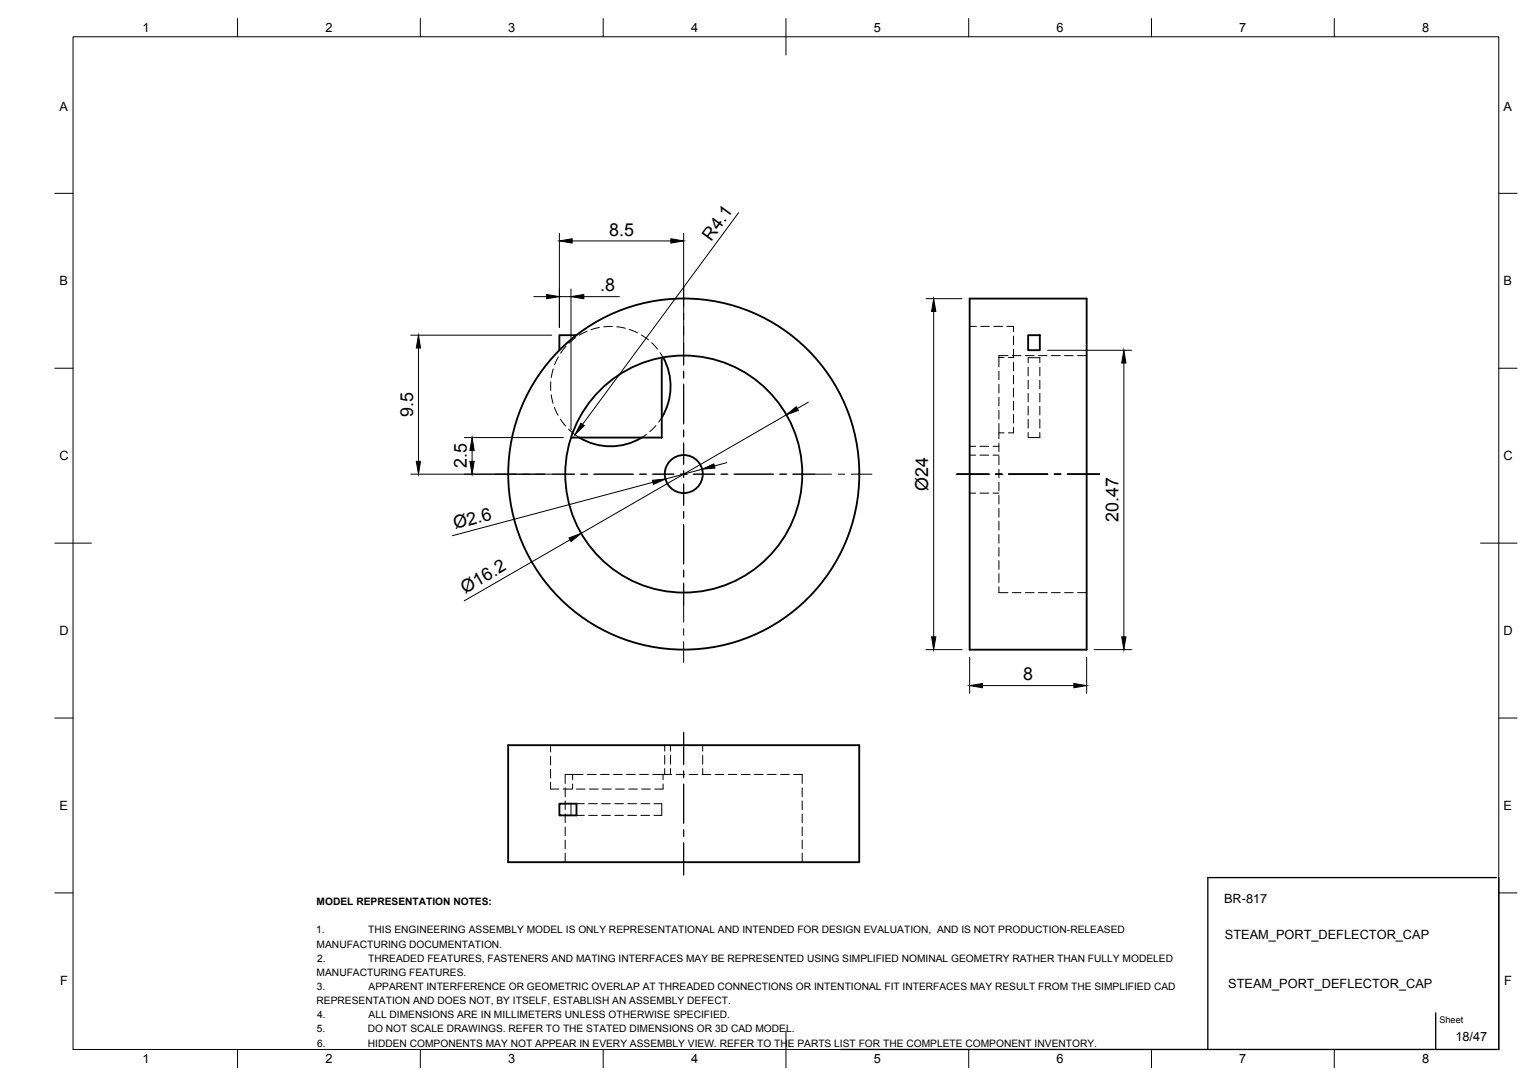
ISO-10303-21;
HEADER;
FILE_DESCRIPTION((''),'2;1');
FILE_NAME('STEAM_PORT_DEFLECTOR_CAP.step','2026-10-01T22:07:29-07:00',(''),(''),'','','');
FILE_SCHEMA (('AUTOMOTIVE_DESIGN { 1 0 10303 214 3 1 1 }'));
ENDSEC;
DATA;
#10=MECHANICAL_DESIGN_GEOMETRIC_PRESENTATION_REPRESENTATION('',(#552),#15484);
#482=SHAPE_REPRESENTATION_RELATIONSHIP('SRR','None',#15631,#517) ;
#517=ADVANCED_BREP_SHAPE_REPRESENTATION('',(#594),#15455) ;
#552=STYLED_ITEM('',(#15836),#594) ;
#594=MANIFOLD_SOLID_BREP('STEAM_PORT_DEFLECTOR_CAP',#8261) ;
#663=CYLINDRICAL_SURFACE('',#8912,0.13) ;
#664=CYLINDRICAL_SURFACE('',#8918,0.41) ;
#665=CYLINDRICAL_SURFACE('',#8922,0.81) ;
#666=CYLINDRICAL_SURFACE('',#8929,1.2) ;
#853=FACE_BOUND('',#2043,.T.) ;
#854=FACE_BOUND('',#2045,.T.) ;
#855=FACE_BOUND('',#2047,.T.) ;
#856=FACE_BOUND('',#2048,.T.) ;
#857=FACE_BOUND('',#2050,.T.) ;
#858=FACE_BOUND('',#2052,.T.) ;
#960=CIRCLE('',#8902,1.2) ;
#961=CIRCLE('',#8905,1.2) ;
#962=CIRCLE('',#8907,0.81) ;
#963=CIRCLE('',#8909,0.81) ;
#964=CIRCLE('',#8913,0.13) ;
#965=CIRCLE('',#8914,0.13) ;
#966=CIRCLE('',#8916,0.81) ;
#967=CIRCLE('',#8917,0.41) ;
#968=CIRCLE('',#8919,0.41) ;
#969=CIRCLE('',#8920,0.41) ;
#970=CIRCLE('',#8921,0.41) ;
#971=CIRCLE('',#8923,0.81) ;
#972=CIRCLE('',#8924,0.81) ;
#973=CIRCLE('',#8925,0.81) ;
#974=CIRCLE('',#8928,1.2) ;
#975=CIRCLE('',#8930,1.2) ;
#1488=FACE_OUTER_BOUND('',#2031,.T.) ;
#1489=FACE_OUTER_BOUND('',#2032,.T.) ;
#1490=FACE_OUTER_BOUND('',#2033,.T.) ;
#1491=FACE_OUTER_BOUND('',#2034,.T.) ;
#1492=FACE_OUTER_BOUND('',#2035,.T.) ;
#1493=FACE_OUTER_BOUND('',#2036,.T.) ;
#1494=FACE_OUTER_BOUND('',#2037,.T.) ;
#1495=FACE_OUTER_BOUND('',#2038,.T.) ;
#1496=FACE_OUTER_BOUND('',#2039,.T.) ;
#1497=FACE_OUTER_BOUND('',#2040,.T.) ;
#1498=FACE_OUTER_BOUND('',#2041,.T.) ;
#1499=FACE_OUTER_BOUND('',#2042,.T.) ;
#1500=FACE_OUTER_BOUND('',#2044,.T.) ;
#1501=FACE_OUTER_BOUND('',#2046,.T.) ;
#1502=FACE_OUTER_BOUND('',#2049,.T.) ;
#1503=FACE_OUTER_BOUND('',#2051,.T.) ;
#2031=EDGE_LOOP('',(#5779,#5780,#5781,#5782)) ;
#2032=EDGE_LOOP('',(#5783,#5784,#5785)) ;
#2033=EDGE_LOOP('',(#5786,#5787,#5788,#5789)) ;
#2034=EDGE_LOOP('',(#5790,#5791,#5792)) ;
#2035=EDGE_LOOP('',(#5793,#5794,#5795)) ;
#2036=EDGE_LOOP('',(#5796,#5797,#5798)) ;
#2037=EDGE_LOOP('',(#5799,#5800,#5801,#5802)) ;
#2038=EDGE_LOOP('',(#5803,#5804,#5805,#5806)) ;
#2039=EDGE_LOOP('',(#5807,#5808,#5809,#5810)) ;
#2040=EDGE_LOOP('',(#5811,#5812)) ;
#2041=EDGE_LOOP('',(#5813,#5814,#5815,#5816,#5817,#5818,#5819,#5820)) ;
#2042=EDGE_LOOP('',(#5821,#5822,#5823,#5824,#5825,#5826,#5827,#5828)) ;
#2043=EDGE_LOOP('',(#5829,#5830,#5831,#5832)) ;
#2044=EDGE_LOOP('',(#5833,#5834,#5835,#5836)) ;
#2045=EDGE_LOOP('',(#5837)) ;
#2046=EDGE_LOOP('',(#5838)) ;
#2047=EDGE_LOOP('',(#5839)) ;
#2048=EDGE_LOOP('',(#5840)) ;
#2049=EDGE_LOOP('',(#5841,#5842,#5843,#5844)) ;
#2050=EDGE_LOOP('',(#5845,#5846,#5847,#5848)) ;
#2051=EDGE_LOOP('',(#5849)) ;
#2052=EDGE_LOOP('',(#5850)) ;
#2618=LINE('',#13453,#3092) ;
#2619=LINE('',#13455,#3093) ;
#2620=LINE('',#13457,#3094) ;
#2621=LINE('',#13458,#3095) ;
#2622=LINE('',#13464,#3096) ;
#2623=LINE('',#13465,#3097) ;
#2624=LINE('',#13468,#3098) ;
#2625=LINE('',#13470,#3099) ;
#2626=LINE('',#13471,#3100) ;
#2627=LINE('',#13475,#3101) ;
#2628=LINE('',#13479,#3102) ;
#2629=LINE('',#13483,#3103) ;
#2630=LINE('',#13485,#3104) ;
#2631=LINE('',#13487,#3105) ;
#2632=LINE('',#13492,#3106) ;
#2633=LINE('',#13501,#3107) ;
#2634=LINE('',#13505,#3108) ;
#2635=LINE('',#13509,#3109) ;
#2636=LINE('',#13514,#3110) ;
#2637=LINE('',#13523,#3111) ;
#3092=VECTOR('',#10541,1.) ;
#3093=VECTOR('',#10542,1.) ;
#3094=VECTOR('',#10543,1.) ;
#3095=VECTOR('',#10544,1.) ;
#3096=VECTOR('',#10549,1.) ;
#3097=VECTOR('',#10550,1.) ;
#3098=VECTOR('',#10553,1.) ;
#3099=VECTOR('',#10554,1.) ;
#3100=VECTOR('',#10555,1.) ;
#3101=VECTOR('',#10560,1.) ;
#3102=VECTOR('',#10565,1.) ;
#3103=VECTOR('',#10570,1.) ;
#3104=VECTOR('',#10573,1.) ;
#3105=VECTOR('',#10576,1.) ;
#3106=VECTOR('',#10581,0.13) ;
#3107=VECTOR('',#10592,1.) ;
#3108=VECTOR('',#10595,0.41) ;
#3109=VECTOR('',#10600,1.) ;
#3110=VECTOR('',#10605,0.81) ;
#3111=VECTOR('',#10618,1.2) ;
#3557=VERTEX_POINT('',#13451) ;
#3558=VERTEX_POINT('',#13452) ;
#3559=VERTEX_POINT('',#13454) ;
#3560=VERTEX_POINT('',#13456) ;
#3561=VERTEX_POINT('',#13460) ;
#3562=VERTEX_POINT('',#13461) ;
#3563=VERTEX_POINT('',#13463) ;
#3564=VERTEX_POINT('',#13467) ;
#3565=VERTEX_POINT('',#13469) ;
#3566=VERTEX_POINT('',#13473) ;
#3567=VERTEX_POINT('',#13477) ;
#3568=VERTEX_POINT('',#13481) ;
#3569=VERTEX_POINT('',#13489) ;
#3570=VERTEX_POINT('',#13491) ;
#3571=VERTEX_POINT('',#13495) ;
#3572=VERTEX_POINT('',#13496) ;
#3573=VERTEX_POINT('',#13500) ;
#3574=VERTEX_POINT('',#13502) ;
#3575=VERTEX_POINT('',#13504) ;
#3576=VERTEX_POINT('',#13507) ;
#3577=VERTEX_POINT('',#13511) ;
#3578=VERTEX_POINT('',#13513) ;
#3579=VERTEX_POINT('',#13519) ;
#3580=VERTEX_POINT('',#13522) ;
#4394=EDGE_CURVE('',#3557,#3558,#2618,.T.) ;
#4395=EDGE_CURVE('',#3559,#3557,#2619,.T.) ;
#4396=EDGE_CURVE('',#3560,#3559,#2620,.T.) ;
#4397=EDGE_CURVE('',#3558,#3560,#2621,.T.) ;
#4398=EDGE_CURVE('',#3561,#3562,#960,.T.) ;
#4399=EDGE_CURVE('',#3561,#3563,#2622,.T.) ;
#4400=EDGE_CURVE('',#3563,#3562,#2623,.T.) ;
#4401=EDGE_CURVE('',#3564,#3561,#2624,.T.) ;
#4402=EDGE_CURVE('',#3565,#3564,#2625,.T.) ;
#4403=EDGE_CURVE('',#3563,#3565,#2626,.T.) ;
#4404=EDGE_CURVE('',#3566,#3564,#961,.T.) ;
#4405=EDGE_CURVE('',#3566,#3565,#2627,.T.) ;
#4406=EDGE_CURVE('',#3567,#3557,#962,.T.) ;
#4407=EDGE_CURVE('',#3567,#3559,#2628,.T.) ;
#4408=EDGE_CURVE('',#3558,#3568,#963,.T.) ;
#4409=EDGE_CURVE('',#3560,#3568,#2629,.T.) ;
#4410=EDGE_CURVE('',#3568,#3567,#2630,.T.) ;
#4411=EDGE_CURVE('',#3562,#3566,#2631,.T.) ;
#4412=EDGE_CURVE('',#3569,#3569,#964,.T.) ;
#4413=EDGE_CURVE('',#3569,#3570,#2632,.T.) ;
#4414=EDGE_CURVE('',#3570,#3570,#965,.T.) ;
#4415=EDGE_CURVE('',#3571,#3572,#966,.T.) ;
#4416=EDGE_CURVE('',#3572,#3571,#967,.T.) ;
#4417=EDGE_CURVE('',#3573,#3571,#2633,.T.) ;
#4418=EDGE_CURVE('',#3574,#3573,#968,.T.) ;
#4419=EDGE_CURVE('',#3574,#3575,#2634,.T.) ;
#4420=EDGE_CURVE('',#3575,#3575,#969,.T.) ;
#4421=EDGE_CURVE('',#3576,#3574,#970,.T.) ;
#4422=EDGE_CURVE('',#3572,#3576,#2635,.T.) ;
#4423=EDGE_CURVE('',#3577,#3577,#971,.T.) ;
#4424=EDGE_CURVE('',#3577,#3578,#2636,.T.) ;
#4425=EDGE_CURVE('',#3573,#3578,#972,.T.) ;
#4426=EDGE_CURVE('',#3578,#3576,#973,.T.) ;
#4427=EDGE_CURVE('',#3579,#3579,#974,.T.) ;
#4428=EDGE_CURVE('',#3579,#3580,#2637,.T.) ;
#4429=EDGE_CURVE('',#3580,#3580,#975,.T.) ;
#5779=ORIENTED_EDGE('',*,*,#4394,.F.) ;
#5780=ORIENTED_EDGE('',*,*,#4395,.F.) ;
#5781=ORIENTED_EDGE('',*,*,#4396,.F.) ;
#5782=ORIENTED_EDGE('',*,*,#4397,.F.) ;
#5783=ORIENTED_EDGE('',*,*,#4398,.F.) ;
#5784=ORIENTED_EDGE('',*,*,#4399,.T.) ;
#5785=ORIENTED_EDGE('',*,*,#4400,.T.) ;
#5786=ORIENTED_EDGE('',*,*,#4401,.F.) ;
#5787=ORIENTED_EDGE('',*,*,#4402,.F.) ;
#5788=ORIENTED_EDGE('',*,*,#4403,.F.) ;
#5789=ORIENTED_EDGE('',*,*,#4399,.F.) ;
#5790=ORIENTED_EDGE('',*,*,#4404,.F.) ;
#5791=ORIENTED_EDGE('',*,*,#4405,.T.) ;
#5792=ORIENTED_EDGE('',*,*,#4402,.T.) ;
#5793=ORIENTED_EDGE('',*,*,#4406,.F.) ;
#5794=ORIENTED_EDGE('',*,*,#4407,.T.) ;
#5795=ORIENTED_EDGE('',*,*,#4395,.T.) ;
#5796=ORIENTED_EDGE('',*,*,#4408,.F.) ;
#5797=ORIENTED_EDGE('',*,*,#4397,.T.) ;
#5798=ORIENTED_EDGE('',*,*,#4409,.T.) ;
#5799=ORIENTED_EDGE('',*,*,#4410,.F.) ;
#5800=ORIENTED_EDGE('',*,*,#4409,.F.) ;
#5801=ORIENTED_EDGE('',*,*,#4396,.T.) ;
#5802=ORIENTED_EDGE('',*,*,#4407,.F.) ;
#5803=ORIENTED_EDGE('',*,*,#4411,.F.) ;
#5804=ORIENTED_EDGE('',*,*,#4400,.F.) ;
#5805=ORIENTED_EDGE('',*,*,#4403,.T.) ;
#5806=ORIENTED_EDGE('',*,*,#4405,.F.) ;
#5807=ORIENTED_EDGE('',*,*,#4412,.F.) ;
#5808=ORIENTED_EDGE('',*,*,#4413,.T.) ;
#5809=ORIENTED_EDGE('',*,*,#4414,.F.) ;
#5810=ORIENTED_EDGE('',*,*,#4413,.F.) ;
#5811=ORIENTED_EDGE('',*,*,#4415,.F.) ;
#5812=ORIENTED_EDGE('',*,*,#4416,.F.) ;
#5813=ORIENTED_EDGE('',*,*,#4417,.F.) ;
#5814=ORIENTED_EDGE('',*,*,#4418,.F.) ;
#5815=ORIENTED_EDGE('',*,*,#4419,.T.) ;
#5816=ORIENTED_EDGE('',*,*,#4420,.F.) ;
#5817=ORIENTED_EDGE('',*,*,#4419,.F.) ;
#5818=ORIENTED_EDGE('',*,*,#4421,.F.) ;
#5819=ORIENTED_EDGE('',*,*,#4422,.F.) ;
#5820=ORIENTED_EDGE('',*,*,#4416,.T.) ;
#5821=ORIENTED_EDGE('',*,*,#4423,.F.) ;
#5822=ORIENTED_EDGE('',*,*,#4424,.T.) ;
#5823=ORIENTED_EDGE('',*,*,#4425,.F.) ;
#5824=ORIENTED_EDGE('',*,*,#4417,.T.) ;
#5825=ORIENTED_EDGE('',*,*,#4415,.T.) ;
#5826=ORIENTED_EDGE('',*,*,#4422,.T.) ;
#5827=ORIENTED_EDGE('',*,*,#4426,.F.) ;
#5828=ORIENTED_EDGE('',*,*,#4424,.F.) ;
#5829=ORIENTED_EDGE('',*,*,#4406,.T.) ;
#5830=ORIENTED_EDGE('',*,*,#4394,.T.) ;
#5831=ORIENTED_EDGE('',*,*,#4408,.T.) ;
#5832=ORIENTED_EDGE('',*,*,#4410,.T.) ;
#5833=ORIENTED_EDGE('',*,*,#4421,.T.) ;
#5834=ORIENTED_EDGE('',*,*,#4418,.T.) ;
#5835=ORIENTED_EDGE('',*,*,#4425,.T.) ;
#5836=ORIENTED_EDGE('',*,*,#4426,.T.) ;
#5837=ORIENTED_EDGE('',*,*,#4412,.T.) ;
#5838=ORIENTED_EDGE('',*,*,#4427,.T.) ;
#5839=ORIENTED_EDGE('',*,*,#4414,.T.) ;
#5840=ORIENTED_EDGE('',*,*,#4420,.T.) ;
#5841=ORIENTED_EDGE('',*,*,#4427,.F.) ;
#5842=ORIENTED_EDGE('',*,*,#4428,.T.) ;
#5843=ORIENTED_EDGE('',*,*,#4429,.F.) ;
#5844=ORIENTED_EDGE('',*,*,#4428,.F.) ;
#5845=ORIENTED_EDGE('',*,*,#4404,.T.) ;
#5846=ORIENTED_EDGE('',*,*,#4401,.T.) ;
#5847=ORIENTED_EDGE('',*,*,#4398,.T.) ;
#5848=ORIENTED_EDGE('',*,*,#4411,.T.) ;
#5849=ORIENTED_EDGE('',*,*,#4429,.T.) ;
#5850=ORIENTED_EDGE('',*,*,#4423,.T.) ;
#7622=PLANE('',#8900) ;
#7623=PLANE('',#8901) ;
#7624=PLANE('',#8903) ;
#7625=PLANE('',#8904) ;
#7626=PLANE('',#8906) ;
#7627=PLANE('',#8908) ;
#7628=PLANE('',#8910) ;
#7629=PLANE('',#8911) ;
#7630=PLANE('',#8915) ;
#7631=PLANE('',#8926) ;
#7632=PLANE('',#8927) ;
#7633=PLANE('',#8931) ;
#7875=ADVANCED_FACE('',(#1488),#7622,.F.) ;
#7876=ADVANCED_FACE('',(#1489),#7623,.T.) ;
#7877=ADVANCED_FACE('',(#1490),#7624,.F.) ;
#7878=ADVANCED_FACE('',(#1491),#7625,.F.) ;
#7879=ADVANCED_FACE('',(#1492),#7626,.F.) ;
#7880=ADVANCED_FACE('',(#1493),#7627,.T.) ;
#7881=ADVANCED_FACE('',(#1494),#7628,.F.) ;
#7882=ADVANCED_FACE('',(#1495),#7629,.F.) ;
#7883=ADVANCED_FACE('',(#1496),#663,.F.) ;
#7884=ADVANCED_FACE('',(#1497),#7630,.F.) ;
#7885=ADVANCED_FACE('',(#1498),#664,.F.) ;
#7886=ADVANCED_FACE('',(#1499,#853),#665,.F.) ;
#7887=ADVANCED_FACE('',(#1500,#854),#7631,.T.) ;
#7888=ADVANCED_FACE('',(#1501,#855,#856),#7632,.T.) ;
#7889=ADVANCED_FACE('',(#1502,#857),#666,.T.) ;
#7890=ADVANCED_FACE('',(#1503,#858),#7633,.T.) ;
#8261=CLOSED_SHELL('',(#7875,#7876,#7877,#7878,#7879,#7880,#7881,#7882,
#7883,#7884,#7885,#7886,#7887,#7888,#7889,#7890)) ;
#8899=AXIS2_PLACEMENT_3D('',#13449,#10537,#10538) ;
#8900=AXIS2_PLACEMENT_3D('',#13450,#10539,#10540) ;
#8901=AXIS2_PLACEMENT_3D('',#13459,#10545,#10546) ;
#8902=AXIS2_PLACEMENT_3D('',#13462,#10547,#10548) ;
#8903=AXIS2_PLACEMENT_3D('',#13466,#10551,#10552) ;
#8904=AXIS2_PLACEMENT_3D('',#13472,#10556,#10557) ;
#8905=AXIS2_PLACEMENT_3D('',#13474,#10558,#10559) ;
#8906=AXIS2_PLACEMENT_3D('',#13476,#10561,#10562) ;
#8907=AXIS2_PLACEMENT_3D('',#13478,#10563,#10564) ;
#8908=AXIS2_PLACEMENT_3D('',#13480,#10566,#10567) ;
#8909=AXIS2_PLACEMENT_3D('',#13482,#10568,#10569) ;
#8910=AXIS2_PLACEMENT_3D('',#13484,#10571,#10572) ;
#8911=AXIS2_PLACEMENT_3D('',#13486,#10574,#10575) ;
#8912=AXIS2_PLACEMENT_3D('',#13488,#10577,#10578) ;
#8913=AXIS2_PLACEMENT_3D('',#13490,#10579,#10580) ;
#8914=AXIS2_PLACEMENT_3D('',#13493,#10582,#10583) ;
#8915=AXIS2_PLACEMENT_3D('',#13494,#10584,#10585) ;
#8916=AXIS2_PLACEMENT_3D('',#13497,#10586,#10587) ;
#8917=AXIS2_PLACEMENT_3D('',#13498,#10588,#10589) ;
#8918=AXIS2_PLACEMENT_3D('',#13499,#10590,#10591) ;
#8919=AXIS2_PLACEMENT_3D('',#13503,#10593,#10594) ;
#8920=AXIS2_PLACEMENT_3D('',#13506,#10596,#10597) ;
#8921=AXIS2_PLACEMENT_3D('',#13508,#10598,#10599) ;
#8922=AXIS2_PLACEMENT_3D('',#13510,#10601,#10602) ;
#8923=AXIS2_PLACEMENT_3D('',#13512,#10603,#10604) ;
#8924=AXIS2_PLACEMENT_3D('',#13515,#10606,#10607) ;
#8925=AXIS2_PLACEMENT_3D('',#13516,#10608,#10609) ;
#8926=AXIS2_PLACEMENT_3D('',#13517,#10610,#10611) ;
#8927=AXIS2_PLACEMENT_3D('',#13518,#10612,#10613) ;
#8928=AXIS2_PLACEMENT_3D('',#13520,#10614,#10615) ;
#8929=AXIS2_PLACEMENT_3D('',#13521,#10616,#10617) ;
#8930=AXIS2_PLACEMENT_3D('',#13524,#10619,#10620) ;
#8931=AXIS2_PLACEMENT_3D('',#13525,#10621,#10622) ;
#10537=DIRECTION('axis',(0.,0.,1.)) ;
#10538=DIRECTION('refdir',(1.,0.,0.)) ;
#10539=DIRECTION('center_axis',(1.,0.,0.)) ;
#10540=DIRECTION('ref_axis',(0.,0.,-1.)) ;
#10541=DIRECTION('',(0.,0.,1.)) ;
#10542=DIRECTION('',(0.,1.,0.)) ;
#10543=DIRECTION('',(0.,0.,-1.)) ;
#10544=DIRECTION('',(0.,-1.,0.)) ;
#10545=DIRECTION('center_axis',(0.,0.,1.)) ;
#10546=DIRECTION('ref_axis',(1.,0.,0.)) ;
#10547=DIRECTION('center_axis',(0.,0.,1.)) ;
#10548=DIRECTION('ref_axis',(1.,0.,0.)) ;
#10549=DIRECTION('',(0.,1.,0.)) ;
#10550=DIRECTION('',(-1.,0.,0.)) ;
#10551=DIRECTION('center_axis',(-1.,0.,0.)) ;
#10552=DIRECTION('ref_axis',(0.,0.,1.)) ;
#10553=DIRECTION('',(0.,0.,1.)) ;
#10554=DIRECTION('',(0.,-1.,0.)) ;
#10555=DIRECTION('',(0.,0.,-1.)) ;
#10556=DIRECTION('center_axis',(0.,0.,1.)) ;
#10557=DIRECTION('ref_axis',(1.,0.,0.)) ;
#10558=DIRECTION('center_axis',(0.,0.,-1.)) ;
#10559=DIRECTION('ref_axis',(1.,0.,0.)) ;
#10560=DIRECTION('',(1.,0.,0.)) ;
#10561=DIRECTION('center_axis',(0.,0.,1.)) ;
#10562=DIRECTION('ref_axis',(1.,0.,0.)) ;
#10563=DIRECTION('center_axis',(0.,0.,1.)) ;
#10564=DIRECTION('ref_axis',(1.,0.,0.)) ;
#10565=DIRECTION('',(-1.,0.,0.)) ;
#10566=DIRECTION('center_axis',(0.,0.,1.)) ;
#10567=DIRECTION('ref_axis',(1.,0.,0.)) ;
#10568=DIRECTION('center_axis',(0.,0.,-1.)) ;
#10569=DIRECTION('ref_axis',(1.,0.,0.)) ;
#10570=DIRECTION('',(1.,0.,0.)) ;
#10571=DIRECTION('center_axis',(0.,1.,0.)) ;
#10572=DIRECTION('ref_axis',(0.,0.,1.)) ;
#10573=DIRECTION('',(0.,0.,-1.)) ;
#10574=DIRECTION('center_axis',(0.,-1.,0.)) ;
#10575=DIRECTION('ref_axis',(0.,0.,-1.)) ;
#10576=DIRECTION('',(0.,0.,-1.)) ;
#10577=DIRECTION('center_axis',(0.,0.,1.)) ;
#10578=DIRECTION('ref_axis',(1.,0.,0.)) ;
#10579=DIRECTION('center_axis',(0.,0.,1.)) ;
#10580=DIRECTION('ref_axis',(1.,0.,0.)) ;
#10581=DIRECTION('',(0.,0.,1.)) ;
#10582=DIRECTION('center_axis',(0.,0.,-1.)) ;
#10583=DIRECTION('ref_axis',(1.,0.,0.)) ;
#10584=DIRECTION('center_axis',(0.,0.,-1.)) ;
#10585=DIRECTION('ref_axis',(-1.,0.,0.)) ;
#10586=DIRECTION('center_axis',(0.,0.,1.)) ;
#10587=DIRECTION('ref_axis',(1.,0.,0.)) ;
#10588=DIRECTION('center_axis',(0.,0.,-1.)) ;
#10589=DIRECTION('ref_axis',(1.,0.,0.)) ;
#10590=DIRECTION('center_axis',(0.,0.,1.)) ;
#10591=DIRECTION('ref_axis',(1.,0.,0.)) ;
#10592=DIRECTION('',(0.,0.,-1.)) ;
#10593=DIRECTION('center_axis',(0.,0.,1.)) ;
#10594=DIRECTION('ref_axis',(1.,0.,0.)) ;
#10595=DIRECTION('',(0.,0.,1.)) ;
#10596=DIRECTION('center_axis',(0.,0.,-1.)) ;
#10597=DIRECTION('ref_axis',(1.,0.,0.)) ;
#10598=DIRECTION('center_axis',(0.,0.,1.)) ;
#10599=DIRECTION('ref_axis',(1.,0.,0.)) ;
#10600=DIRECTION('',(0.,0.,1.)) ;
#10601=DIRECTION('center_axis',(0.,0.,1.)) ;
#10602=DIRECTION('ref_axis',(1.,0.,0.)) ;
#10603=DIRECTION('center_axis',(0.,0.,1.)) ;
#10604=DIRECTION('ref_axis',(1.,0.,0.)) ;
#10605=DIRECTION('',(0.,0.,1.)) ;
#10606=DIRECTION('center_axis',(0.,0.,-1.)) ;
#10607=DIRECTION('ref_axis',(1.,0.,0.)) ;
#10608=DIRECTION('center_axis',(0.,0.,-1.)) ;
#10609=DIRECTION('ref_axis',(1.,0.,0.)) ;
#10610=DIRECTION('center_axis',(0.,0.,-1.)) ;
#10611=DIRECTION('ref_axis',(-1.,0.,0.)) ;
#10612=DIRECTION('center_axis',(0.,0.,1.)) ;
#10613=DIRECTION('ref_axis',(1.,0.,0.)) ;
#10614=DIRECTION('center_axis',(0.,0.,1.)) ;
#10615=DIRECTION('ref_axis',(1.,0.,0.)) ;
#10616=DIRECTION('center_axis',(0.,0.,1.)) ;
#10617=DIRECTION('ref_axis',(1.,0.,0.)) ;
#10618=DIRECTION('',(0.,0.,-1.)) ;
#10619=DIRECTION('center_axis',(0.,0.,-1.)) ;
#10620=DIRECTION('ref_axis',(1.,0.,0.)) ;
#10621=DIRECTION('center_axis',(0.,0.,-1.)) ;
#10622=DIRECTION('ref_axis',(-1.,0.,0.)) ;
#13449=CARTESIAN_POINT('',(0.,0.,0.)) ;
#13450=CARTESIAN_POINT('Origin',(2.15,1.4,1.56)) ;
#13451=CARTESIAN_POINT('',(2.15,1.5959899496853,1.52)) ;
#13452=CARTESIAN_POINT('',(2.15,1.5959899496853,1.6)) ;
#13453=CARTESIAN_POINT('',(2.15,1.5959899496853,1.5)) ;
#13454=CARTESIAN_POINT('',(2.15,1.05,1.52)) ;
#13455=CARTESIAN_POINT('',(2.15,1.4,1.52)) ;
#13456=CARTESIAN_POINT('',(2.15,1.05,1.6)) ;
#13457=CARTESIAN_POINT('',(2.15,1.05,1.56)) ;
#13458=CARTESIAN_POINT('',(2.15,1.4,1.6)) ;
#13459=CARTESIAN_POINT('Origin',(2.5,1.4,1.6)) ;
#13460=CARTESIAN_POINT('',(2.85,1.64705371730487,1.6)) ;
#13461=CARTESIAN_POINT('',(2.73314391493076,1.75,1.6)) ;
#13462=CARTESIAN_POINT('Origin',(2.,0.8,1.6)) ;
#13463=CARTESIAN_POINT('',(2.85,1.75,1.6)) ;
#13464=CARTESIAN_POINT('',(2.85,1.4,1.6)) ;
#13465=CARTESIAN_POINT('',(2.5,1.75,1.6)) ;
#13466=CARTESIAN_POINT('Origin',(2.85,1.4,1.56)) ;
#13467=CARTESIAN_POINT('',(2.85,1.64705371730487,1.52)) ;
#13468=CARTESIAN_POINT('',(2.85,1.64705371730487,1.5)) ;
#13469=CARTESIAN_POINT('',(2.85,1.75,1.52)) ;
#13470=CARTESIAN_POINT('',(2.85,1.4,1.52)) ;
#13471=CARTESIAN_POINT('',(2.85,1.75,1.56)) ;
#13472=CARTESIAN_POINT('Origin',(2.5,1.4,1.52)) ;
#13473=CARTESIAN_POINT('',(2.73314391493076,1.75,1.52)) ;
#13474=CARTESIAN_POINT('Origin',(2.,0.8,1.52)) ;
#13475=CARTESIAN_POINT('',(2.5,1.75,1.52)) ;
#13476=CARTESIAN_POINT('Origin',(2.5,1.4,1.52)) ;
#13477=CARTESIAN_POINT('',(2.77045441137033,1.05,1.52)) ;
#13478=CARTESIAN_POINT('Origin',(2.,0.8,1.52)) ;
#13479=CARTESIAN_POINT('',(2.5,1.05,1.52)) ;
#13480=CARTESIAN_POINT('Origin',(2.5,1.4,1.6)) ;
#13481=CARTESIAN_POINT('',(2.77045441137033,1.05,1.6)) ;
#13482=CARTESIAN_POINT('Origin',(2.,0.8,1.6)) ;
#13483=CARTESIAN_POINT('',(2.5,1.05,1.6)) ;
#13484=CARTESIAN_POINT('Origin',(2.5,1.05,1.56)) ;
#13485=CARTESIAN_POINT('',(2.77045441137033,1.05,1.5)) ;
#13486=CARTESIAN_POINT('Origin',(2.5,1.75,1.56)) ;
#13487=CARTESIAN_POINT('',(2.73314391493076,1.75,1.5)) ;
#13488=CARTESIAN_POINT('Origin',(2.,0.8,1.9)) ;
#13489=CARTESIAN_POINT('',(1.87,0.8,1.8)) ;
#13490=CARTESIAN_POINT('Origin',(2.,0.8,1.8)) ;
#13491=CARTESIAN_POINT('',(1.87,0.8,2.)) ;
#13492=CARTESIAN_POINT('',(1.87,0.8,1.9)) ;
#13493=CARTESIAN_POINT('Origin',(2.,0.8,2.)) ;
#13494=CARTESIAN_POINT('Origin',(2.5,1.4,1.7)) ;
#13495=CARTESIAN_POINT('',(2.75920310052949,1.08233074955876,1.7)) ;
#13496=CARTESIAN_POINT('',(2.14079689947051,1.59766925044124,1.7)) ;
#13497=CARTESIAN_POINT('Origin',(2.,0.8,1.7)) ;
#13498=CARTESIAN_POINT('Origin',(2.5,1.4,1.7)) ;
#13499=CARTESIAN_POINT('Origin',(2.5,1.4,1.9)) ;
#13500=CARTESIAN_POINT('',(2.75920310052949,1.08233074955876,1.8)) ;
#13501=CARTESIAN_POINT('',(2.75920310052949,1.08233074955876,1.9)) ;
#13502=CARTESIAN_POINT('',(2.09,1.4,1.8)) ;
#13503=CARTESIAN_POINT('Origin',(2.5,1.4,1.8)) ;
#13504=CARTESIAN_POINT('',(2.09,1.4,2.)) ;
#13505=CARTESIAN_POINT('',(2.09,1.4,1.9)) ;
#13506=CARTESIAN_POINT('Origin',(2.5,1.4,2.)) ;
#13507=CARTESIAN_POINT('',(2.14079689947051,1.59766925044124,1.8)) ;
#13508=CARTESIAN_POINT('Origin',(2.5,1.4,1.8)) ;
#13509=CARTESIAN_POINT('',(2.14079689947051,1.59766925044124,1.9)) ;
#13510=CARTESIAN_POINT('Origin',(2.,0.8,1.5)) ;
#13511=CARTESIAN_POINT('',(1.19,0.8,1.2)) ;
#13512=CARTESIAN_POINT('Origin',(2.,0.8,1.2)) ;
#13513=CARTESIAN_POINT('',(1.19,0.8,1.8)) ;
#13514=CARTESIAN_POINT('',(1.19,0.8,1.5)) ;
#13515=CARTESIAN_POINT('Origin',(2.,0.8,1.8)) ;
#13516=CARTESIAN_POINT('Origin',(2.,0.8,1.8)) ;
#13517=CARTESIAN_POINT('Origin',(2.,0.8,1.8)) ;
#13518=CARTESIAN_POINT('Origin',(2.,0.8,2.)) ;
#13519=CARTESIAN_POINT('',(0.8,0.8,2.)) ;
#13520=CARTESIAN_POINT('Origin',(2.,0.8,2.)) ;
#13521=CARTESIAN_POINT('Origin',(2.,0.8,1.5)) ;
#13522=CARTESIAN_POINT('',(0.8,0.8,1.2)) ;
#13523=CARTESIAN_POINT('',(0.8,0.8,1.5)) ;
#13524=CARTESIAN_POINT('Origin',(2.,0.8,1.2)) ;
#13525=CARTESIAN_POINT('Origin',(2.,0.8,1.2)) ;
#15412=UNCERTAINTY_MEASURE_WITH_UNIT(LENGTH_MEASURE(0.001),#15485,
'DISTANCE_ACCURACY_VALUE',
'Maximum model space distance between geometric entities at asserted c
onnectivities') ;
#15441=UNCERTAINTY_MEASURE_WITH_UNIT(LENGTH_MEASURE(0.001),#15485,
'DISTANCE_ACCURACY_VALUE',
'Maximum model space distance between geometric entities at asserted c
onnectivities') ;
#15455=(
GEOMETRIC_REPRESENTATION_CONTEXT(3)
GLOBAL_UNCERTAINTY_ASSIGNED_CONTEXT((#15412))
GLOBAL_UNIT_ASSIGNED_CONTEXT((#15485,#15487,#15488))
REPRESENTATION_CONTEXT('','3D')
) ;
#15484=(
GEOMETRIC_REPRESENTATION_CONTEXT(3)
GLOBAL_UNCERTAINTY_ASSIGNED_CONTEXT((#15441))
GLOBAL_UNIT_ASSIGNED_CONTEXT((#15485,#15487,#15488))
REPRESENTATION_CONTEXT('','3D')
) ;
#15485=(
LENGTH_UNIT()
NAMED_UNIT(*)
SI_UNIT(.CENTI.,.METRE.)
) ;
#15487=(
NAMED_UNIT(*)
PLANE_ANGLE_UNIT()
SI_UNIT($,.RADIAN.)
) ;
#15488=(
NAMED_UNIT(*)
SI_UNIT($,.STERADIAN.)
SOLID_ANGLE_UNIT()
) ;
#15502=SHAPE_DEFINITION_REPRESENTATION(#15550,#15631) ;
#15550=PRODUCT_DEFINITION_SHAPE('',$,#15674) ;
#15631=SHAPE_REPRESENTATION('',(#8899),#15455) ;
#15660=PRODUCT_DEFINITION_CONTEXT('part definition',#15788,'design') ;
#15674=PRODUCT_DEFINITION('STEAM_PORT_DEFLECTOR_CAP',
'STEAM_PORT_DEFLECTOR_CAP',#15716,#15660) ;
#15716=PRODUCT_DEFINITION_FORMATION('',$,#15803) ;
#15788=APPLICATION_CONTEXT(
'Core Data for Automotive Mechanical Design Process') ;
#15789=PRODUCT_CONTEXT('part definition',#15788,'mechanical') ;
#15803=PRODUCT('STEAM_PORT_DEFLECTOR_CAP','STEAM_PORT_DEFLECTOR_CAP',$,(#15789)) ;
#15836=PRESENTATION_STYLE_ASSIGNMENT((#15848)) ;
#15848=SURFACE_STYLE_USAGE(.BOTH.,#15860) ;
#15860=SURFACE_SIDE_STYLE('',(#15872)) ;
#15872=SURFACE_STYLE_FILL_AREA(#15884) ;
#15884=FILL_AREA_STYLE('Surface - Matte',(#15896)) ;
#15896=FILL_AREA_STYLE_COLOUR('Surface - Matte',#15908) ;
#15908=COLOUR_RGB('Surface - Matte', 0.08235294, 0.09019608, 0.10196078) ;
ENDSEC;
END-ISO-10303-21;
